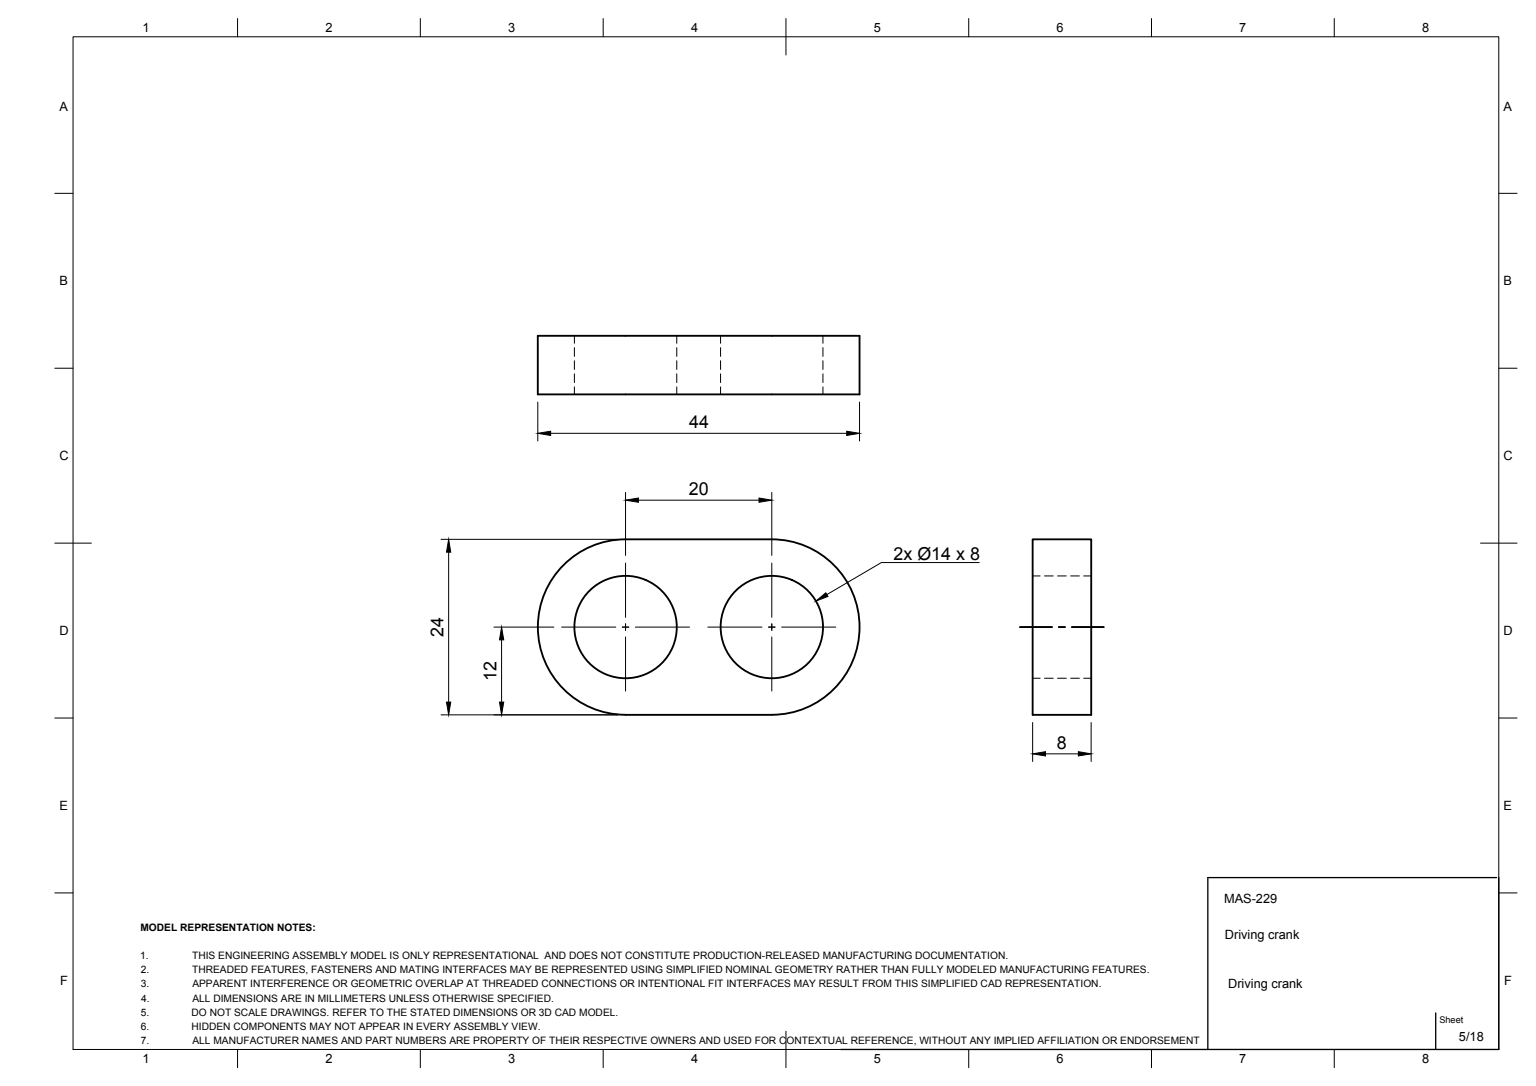
ISO-10303-21;
HEADER;
/* Generated by software containing ST-Developer
 * from STEP Tools, Inc. (www.steptools.com) 
 */

FILE_DESCRIPTION(
/* description */ ('Independently dimensioned six-bar single-leg walking-linkage demonstr
ator. Whole-mm20 crank,60 upper rocker,80/120 ternary coupler,120 lowe
r rocker,140 knee pitch and260 toe reach; ground pivots0/0,60/0,40/60.
 Seven native revolutes close both loops. Four reused native library f
amilies, fully retained shared pins and layered real spacer stacks, bo
nded rubber toe. Benchtop reference mechanism; no complete vehicle, lo
ad, gait stability, adhesive, weld, fit or life rating.'),
/* implementation_level */ '2;1');

FILE_NAME(
/* name */ 'Driving crank.step',
/* time_stamp */ '2026-11-09T20:33:14-08:00',
/* author */ (''),
/* organization */ (''),
/* preprocessor_version */ 'ST-DEVELOPER v20.2',
/* originating_system */ 'Autodesk Translation Framework v15.17.0.0',
/* authorisation */ '');

FILE_SCHEMA (('AUTOMOTIVE_DESIGN { 1 0 10303 214 3 1 1 }'));
ENDSEC;

DATA;
#10=MECHANICAL_DESIGN_GEOMETRIC_PRESENTATION_REPRESENTATION('',(#257),#4048);
#221=SHAPE_REPRESENTATION_RELATIONSHIP('SRR','None',#4145,#239);
#239=ADVANCED_BREP_SHAPE_REPRESENTATION('',(#275),#4032);
#257=STYLED_ITEM('',(#4244),#275);
#275=MANIFOLD_SOLID_BREP('Body1',#2146);
#305=FACE_BOUND('',#583,.T.);
#306=FACE_BOUND('',#584,.T.);
#307=FACE_BOUND('',#586,.T.);
#308=FACE_BOUND('',#587,.T.);
#362=PLANE('',#2406);
#363=PLANE('',#2410);
#364=PLANE('',#2414);
#365=PLANE('',#2415);
#436=FACE_OUTER_BOUND('',#576,.T.);
#437=FACE_OUTER_BOUND('',#577,.T.);
#438=FACE_OUTER_BOUND('',#578,.T.);
#439=FACE_OUTER_BOUND('',#579,.T.);
#440=FACE_OUTER_BOUND('',#580,.T.);
#441=FACE_OUTER_BOUND('',#581,.T.);
#442=FACE_OUTER_BOUND('',#582,.T.);
#443=FACE_OUTER_BOUND('',#585,.T.);
#576=EDGE_LOOP('',(#1587,#1588,#1589,#1590));
#577=EDGE_LOOP('',(#1591,#1592,#1593,#1594));
#578=EDGE_LOOP('',(#1595,#1596,#1597,#1598));
#579=EDGE_LOOP('',(#1599,#1600,#1601,#1602));
#580=EDGE_LOOP('',(#1603,#1604,#1605,#1606));
#581=EDGE_LOOP('',(#1607,#1608,#1609,#1610));
#582=EDGE_LOOP('',(#1611,#1612,#1613,#1614));
#583=EDGE_LOOP('',(#1615));
#584=EDGE_LOOP('',(#1616));
#585=EDGE_LOOP('',(#1617,#1618,#1619,#1620));
#586=EDGE_LOOP('',(#1621));
#587=EDGE_LOOP('',(#1622));
#761=LINE('',#3530,#886);
#762=LINE('',#3536,#887);
#763=LINE('',#3541,#888);
#764=LINE('',#3543,#889);
#765=LINE('',#3545,#890);
#766=LINE('',#3546,#891);
#767=LINE('',#3552,#892);
#768=LINE('',#3555,#893);
#769=LINE('',#3557,#894);
#770=LINE('',#3558,#895);
#886=VECTOR('',#2790,7.);
#887=VECTOR('',#2797,7.);
#888=VECTOR('',#2802,10.);
#889=VECTOR('',#2803,10.);
#890=VECTOR('',#2804,10.);
#891=VECTOR('',#2805,10.);
#892=VECTOR('',#2812,10.);
#893=VECTOR('',#2815,10.);
#894=VECTOR('',#2816,10.);
#895=VECTOR('',#2817,10.);
#988=CIRCLE('',#2401,7.);
#989=CIRCLE('',#2402,7.);
#990=CIRCLE('',#2404,7.);
#991=CIRCLE('',#2405,7.);
#992=CIRCLE('',#2408,12.);
#993=CIRCLE('',#2409,12.);
#994=CIRCLE('',#2412,12.);
#995=CIRCLE('',#2413,12.);
#1122=VERTEX_POINT('',#3527);
#1123=VERTEX_POINT('',#3529);
#1124=VERTEX_POINT('',#3533);
#1125=VERTEX_POINT('',#3535);
#1126=VERTEX_POINT('',#3539);
#1127=VERTEX_POINT('',#3540);
#1128=VERTEX_POINT('',#3542);
#1129=VERTEX_POINT('',#3544);
#1130=VERTEX_POINT('',#3548);
#1131=VERTEX_POINT('',#3550);
#1132=VERTEX_POINT('',#3554);
#1133=VERTEX_POINT('',#3556);
#1297=EDGE_CURVE('',#1122,#1122,#988,.T.);
#1298=EDGE_CURVE('',#1122,#1123,#761,.T.);
#1299=EDGE_CURVE('',#1123,#1123,#989,.T.);
#1300=EDGE_CURVE('',#1124,#1124,#990,.T.);
#1301=EDGE_CURVE('',#1124,#1125,#762,.T.);
#1302=EDGE_CURVE('',#1125,#1125,#991,.T.);
#1303=EDGE_CURVE('',#1126,#1127,#763,.T.);
#1304=EDGE_CURVE('',#1127,#1128,#764,.T.);
#1305=EDGE_CURVE('',#1129,#1128,#765,.T.);
#1306=EDGE_CURVE('',#1126,#1129,#766,.T.);
#1307=EDGE_CURVE('',#1130,#1126,#992,.T.);
#1308=EDGE_CURVE('',#1131,#1129,#993,.T.);
#1309=EDGE_CURVE('',#1130,#1131,#767,.T.);
#1310=EDGE_CURVE('',#1132,#1130,#768,.T.);
#1311=EDGE_CURVE('',#1133,#1131,#769,.T.);
#1312=EDGE_CURVE('',#1132,#1133,#770,.T.);
#1313=EDGE_CURVE('',#1127,#1132,#994,.T.);
#1314=EDGE_CURVE('',#1128,#1133,#995,.T.);
#1587=ORIENTED_EDGE('',*,*,#1297,.F.);
#1588=ORIENTED_EDGE('',*,*,#1298,.T.);
#1589=ORIENTED_EDGE('',*,*,#1299,.F.);
#1590=ORIENTED_EDGE('',*,*,#1298,.F.);
#1591=ORIENTED_EDGE('',*,*,#1300,.F.);
#1592=ORIENTED_EDGE('',*,*,#1301,.T.);
#1593=ORIENTED_EDGE('',*,*,#1302,.F.);
#1594=ORIENTED_EDGE('',*,*,#1301,.F.);
#1595=ORIENTED_EDGE('',*,*,#1303,.T.);
#1596=ORIENTED_EDGE('',*,*,#1304,.T.);
#1597=ORIENTED_EDGE('',*,*,#1305,.F.);
#1598=ORIENTED_EDGE('',*,*,#1306,.F.);
#1599=ORIENTED_EDGE('',*,*,#1307,.T.);
#1600=ORIENTED_EDGE('',*,*,#1306,.T.);
#1601=ORIENTED_EDGE('',*,*,#1308,.F.);
#1602=ORIENTED_EDGE('',*,*,#1309,.F.);
#1603=ORIENTED_EDGE('',*,*,#1310,.T.);
#1604=ORIENTED_EDGE('',*,*,#1309,.T.);
#1605=ORIENTED_EDGE('',*,*,#1311,.F.);
#1606=ORIENTED_EDGE('',*,*,#1312,.F.);
#1607=ORIENTED_EDGE('',*,*,#1313,.T.);
#1608=ORIENTED_EDGE('',*,*,#1312,.T.);
#1609=ORIENTED_EDGE('',*,*,#1314,.F.);
#1610=ORIENTED_EDGE('',*,*,#1304,.F.);
#1611=ORIENTED_EDGE('',*,*,#1314,.T.);
#1612=ORIENTED_EDGE('',*,*,#1311,.T.);
#1613=ORIENTED_EDGE('',*,*,#1308,.T.);
#1614=ORIENTED_EDGE('',*,*,#1305,.T.);
#1615=ORIENTED_EDGE('',*,*,#1297,.T.);
#1616=ORIENTED_EDGE('',*,*,#1300,.T.);
#1617=ORIENTED_EDGE('',*,*,#1313,.F.);
#1618=ORIENTED_EDGE('',*,*,#1303,.F.);
#1619=ORIENTED_EDGE('',*,*,#1307,.F.);
#1620=ORIENTED_EDGE('',*,*,#1310,.F.);
#1621=ORIENTED_EDGE('',*,*,#1299,.T.);
#1622=ORIENTED_EDGE('',*,*,#1302,.T.);
#1970=CYLINDRICAL_SURFACE('',#2400,7.);
#1971=CYLINDRICAL_SURFACE('',#2403,7.);
#1972=CYLINDRICAL_SURFACE('',#2407,12.);
#1973=CYLINDRICAL_SURFACE('',#2411,12.);
#2039=ADVANCED_FACE('',(#436),#1970,.F.);
#2040=ADVANCED_FACE('',(#437),#1971,.F.);
#2041=ADVANCED_FACE('',(#438),#362,.T.);
#2042=ADVANCED_FACE('',(#439),#1972,.T.);
#2043=ADVANCED_FACE('',(#440),#363,.T.);
#2044=ADVANCED_FACE('',(#441),#1973,.T.);
#2045=ADVANCED_FACE('',(#442,#305,#306),#364,.T.);
#2046=ADVANCED_FACE('',(#443,#307,#308),#365,.F.);
#2146=CLOSED_SHELL('',(#2039,#2040,#2041,#2042,#2043,#2044,#2045,#2046));
#2399=AXIS2_PLACEMENT_3D('',#3525,#2784,#2785);
#2400=AXIS2_PLACEMENT_3D('',#3526,#2786,#2787);
#2401=AXIS2_PLACEMENT_3D('',#3528,#2788,#2789);
#2402=AXIS2_PLACEMENT_3D('',#3531,#2791,#2792);
#2403=AXIS2_PLACEMENT_3D('',#3532,#2793,#2794);
#2404=AXIS2_PLACEMENT_3D('',#3534,#2795,#2796);
#2405=AXIS2_PLACEMENT_3D('',#3537,#2798,#2799);
#2406=AXIS2_PLACEMENT_3D('',#3538,#2800,#2801);
#2407=AXIS2_PLACEMENT_3D('',#3547,#2806,#2807);
#2408=AXIS2_PLACEMENT_3D('',#3549,#2808,#2809);
#2409=AXIS2_PLACEMENT_3D('',#3551,#2810,#2811);
#2410=AXIS2_PLACEMENT_3D('',#3553,#2813,#2814);
#2411=AXIS2_PLACEMENT_3D('',#3559,#2818,#2819);
#2412=AXIS2_PLACEMENT_3D('',#3560,#2820,#2821);
#2413=AXIS2_PLACEMENT_3D('',#3561,#2822,#2823);
#2414=AXIS2_PLACEMENT_3D('',#3562,#2824,#2825);
#2415=AXIS2_PLACEMENT_3D('',#3563,#2826,#2827);
#2784=DIRECTION('axis',(0.,0.,1.));
#2785=DIRECTION('refdir',(1.,0.,0.));
#2786=DIRECTION('center_axis',(0.,0.,-1.));
#2787=DIRECTION('ref_axis',(1.,0.,0.));
#2788=DIRECTION('center_axis',(0.,0.,-1.));
#2789=DIRECTION('ref_axis',(1.,0.,0.));
#2790=DIRECTION('',(0.,0.,-1.));
#2791=DIRECTION('center_axis',(0.,0.,1.));
#2792=DIRECTION('ref_axis',(1.,0.,0.));
#2793=DIRECTION('center_axis',(0.,0.,-1.));
#2794=DIRECTION('ref_axis',(1.,0.,0.));
#2795=DIRECTION('center_axis',(0.,0.,-1.));
#2796=DIRECTION('ref_axis',(1.,0.,0.));
#2797=DIRECTION('',(0.,0.,-1.));
#2798=DIRECTION('center_axis',(0.,0.,1.));
#2799=DIRECTION('ref_axis',(1.,0.,0.));
#2800=DIRECTION('center_axis',(0.,1.,0.));
#2801=DIRECTION('ref_axis',(-1.,0.,0.));
#2802=DIRECTION('',(-1.,0.,0.));
#2803=DIRECTION('',(0.,0.,1.));
#2804=DIRECTION('',(-1.,0.,0.));
#2805=DIRECTION('',(0.,0.,1.));
#2806=DIRECTION('center_axis',(0.,0.,1.));
#2807=DIRECTION('ref_axis',(0.,-1.,0.));
#2808=DIRECTION('center_axis',(0.,0.,1.));
#2809=DIRECTION('ref_axis',(0.,-1.,0.));
#2810=DIRECTION('center_axis',(0.,0.,1.));
#2811=DIRECTION('ref_axis',(0.,-1.,0.));
#2812=DIRECTION('',(0.,0.,1.));
#2813=DIRECTION('center_axis',(0.,-1.,0.));
#2814=DIRECTION('ref_axis',(1.,0.,0.));
#2815=DIRECTION('',(1.,0.,0.));
#2816=DIRECTION('',(1.,0.,0.));
#2817=DIRECTION('',(0.,0.,1.));
#2818=DIRECTION('center_axis',(0.,0.,1.));
#2819=DIRECTION('ref_axis',(0.,1.,0.));
#2820=DIRECTION('center_axis',(0.,0.,1.));
#2821=DIRECTION('ref_axis',(0.,1.,0.));
#2822=DIRECTION('center_axis',(0.,0.,1.));
#2823=DIRECTION('ref_axis',(0.,1.,0.));
#2824=DIRECTION('center_axis',(0.,0.,1.));
#2825=DIRECTION('ref_axis',(1.,0.,0.));
#2826=DIRECTION('center_axis',(0.,0.,1.));
#2827=DIRECTION('ref_axis',(1.,0.,0.));
#3525=CARTESIAN_POINT('',(0.,0.,0.));
#3526=CARTESIAN_POINT('Origin',(0.,0.,4.));
#3527=CARTESIAN_POINT('',(-7.,8.57252759403147E-16,8.));
#3528=CARTESIAN_POINT('Origin',(0.,0.,8.));
#3529=CARTESIAN_POINT('',(-7.,8.57252759403147E-16,0.));
#3530=CARTESIAN_POINT('',(-7.,8.57252759403147E-16,4.));
#3531=CARTESIAN_POINT('Origin',(0.,0.,0.));
#3532=CARTESIAN_POINT('Origin',(20.,0.,4.));
#3533=CARTESIAN_POINT('',(13.,8.57252759403147E-16,8.));
#3534=CARTESIAN_POINT('Origin',(20.,0.,8.));
#3535=CARTESIAN_POINT('',(13.,8.57252759403147E-16,0.));
#3536=CARTESIAN_POINT('',(13.,8.57252759403147E-16,4.));
#3537=CARTESIAN_POINT('Origin',(20.,0.,0.));
#3538=CARTESIAN_POINT('Origin',(20.,12.,0.));
#3539=CARTESIAN_POINT('',(20.,12.,0.));
#3540=CARTESIAN_POINT('',(0.,12.,0.));
#3541=CARTESIAN_POINT('',(20.,12.,0.));
#3542=CARTESIAN_POINT('',(0.,12.,8.));
#3543=CARTESIAN_POINT('',(0.,12.,0.));
#3544=CARTESIAN_POINT('',(20.,12.,8.));
#3545=CARTESIAN_POINT('',(20.,12.,8.));
#3546=CARTESIAN_POINT('',(20.,12.,0.));
#3547=CARTESIAN_POINT('Origin',(20.,0.,0.));
#3548=CARTESIAN_POINT('',(20.,-12.,0.));
#3549=CARTESIAN_POINT('Origin',(20.,0.,0.));
#3550=CARTESIAN_POINT('',(20.,-12.,8.));
#3551=CARTESIAN_POINT('Origin',(20.,0.,8.));
#3552=CARTESIAN_POINT('',(20.,-12.,0.));
#3553=CARTESIAN_POINT('Origin',(0.,-12.,0.));
#3554=CARTESIAN_POINT('',(-1.46957615897682E-15,-12.,0.));
#3555=CARTESIAN_POINT('',(0.,-12.,0.));
#3556=CARTESIAN_POINT('',(-1.46957615897682E-15,-12.,8.));
#3557=CARTESIAN_POINT('',(0.,-12.,8.));
#3558=CARTESIAN_POINT('',(-1.46957615897682E-15,-12.,0.));
#3559=CARTESIAN_POINT('Origin',(0.,0.,0.));
#3560=CARTESIAN_POINT('Origin',(0.,0.,0.));
#3561=CARTESIAN_POINT('Origin',(0.,0.,8.));
#3562=CARTESIAN_POINT('Origin',(10.,0.,8.));
#3563=CARTESIAN_POINT('Origin',(10.,0.,0.));
#4012=UNCERTAINTY_MEASURE_WITH_UNIT(LENGTH_MEASURE(0.01),#4049,
'DISTANCE_ACCURACY_VALUE',
'Maximum model space distance between geometric entities at asserted c
onnectivities');
#4028=UNCERTAINTY_MEASURE_WITH_UNIT(LENGTH_MEASURE(0.01),#4049,
'DISTANCE_ACCURACY_VALUE',
'Maximum model space distance between geometric entities at asserted c
onnectivities');
#4032=(
GEOMETRIC_REPRESENTATION_CONTEXT(3)
GLOBAL_UNCERTAINTY_ASSIGNED_CONTEXT((#4012))
GLOBAL_UNIT_ASSIGNED_CONTEXT((#4049,#4051,#4052))
REPRESENTATION_CONTEXT('','3D')
);
#4048=(
GEOMETRIC_REPRESENTATION_CONTEXT(3)
GLOBAL_UNCERTAINTY_ASSIGNED_CONTEXT((#4028))
GLOBAL_UNIT_ASSIGNED_CONTEXT((#4049,#4051,#4052))
REPRESENTATION_CONTEXT('','3D')
);
#4049=(
LENGTH_UNIT()
NAMED_UNIT(*)
SI_UNIT(.MILLI.,.METRE.)
);
#4051=(
NAMED_UNIT(*)
PLANE_ANGLE_UNIT()
SI_UNIT($,.RADIAN.)
);
#4052=(
NAMED_UNIT(*)
SI_UNIT($,.STERADIAN.)
SOLID_ANGLE_UNIT()
);
#4056=SHAPE_DEFINITION_REPRESENTATION(#4075,#4145);
#4075=PRODUCT_DEFINITION_SHAPE('',$,#4165);
#4145=SHAPE_REPRESENTATION('',(#2399),#4032);
#4161=PRODUCT_DEFINITION_CONTEXT('part definition',#4220,'design');
#4165=PRODUCT_DEFINITION('Driving crank','Driving crank',#4184,#4161);
#4184=PRODUCT_DEFINITION_FORMATION('',$,#4225);
#4220=APPLICATION_CONTEXT(
'Core Data for Automotive Mechanical Design Process');
#4221=PRODUCT_CONTEXT('part definition',#4220,'mechanical');
#4225=PRODUCT('Driving crank','Driving crank','Driving crank',(#4221));
#4244=PRESENTATION_STYLE_ASSIGNMENT((#4258));
#4258=SURFACE_STYLE_USAGE(.BOTH.,#4272);
#4272=SURFACE_SIDE_STYLE('',(#4286));
#4286=SURFACE_STYLE_FILL_AREA(#4300);
#4300=FILL_AREA_STYLE('Driving crank finish',(#4314));
#4314=FILL_AREA_STYLE_COLOUR('Driving crank finish',#4328);
#4328=COLOUR_RGB('Driving crank finish',0.0901960784313725,0.270588235294118,
0.513725490196078);
ENDSEC;
END-ISO-10303-21;
